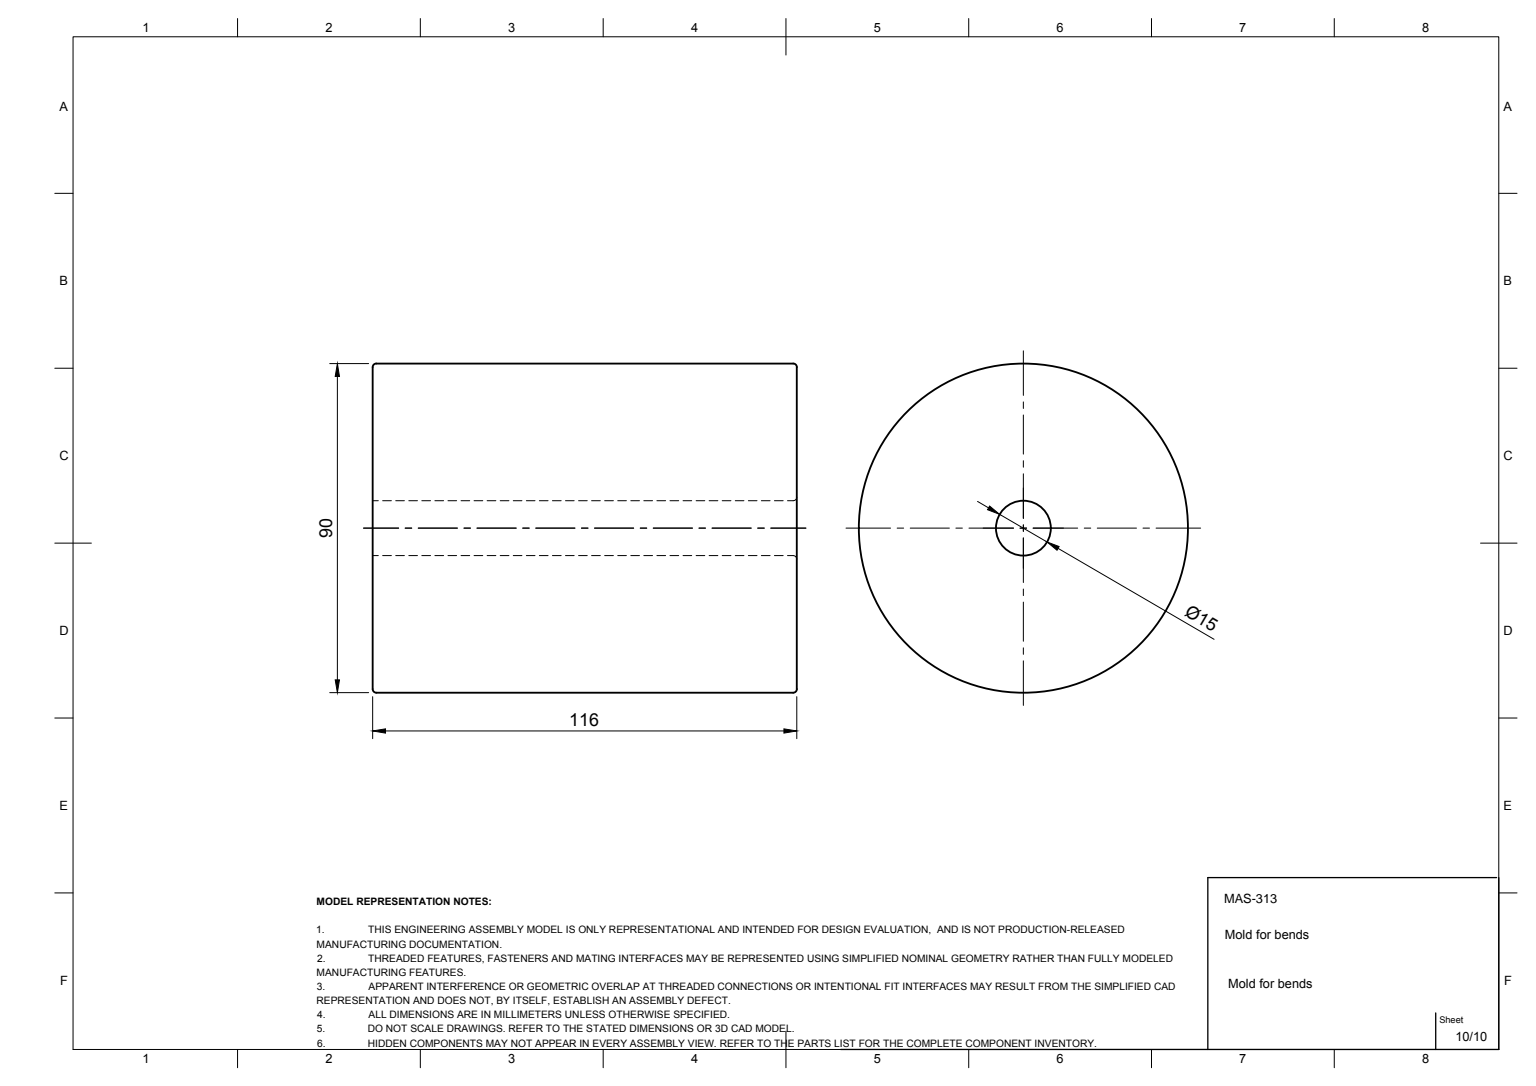
ISO-10303-21;
HEADER;
FILE_DESCRIPTION (('STEP AP214'),
    '1' );
FILE_NAME ('Mold for bends.step',
    '2026-10-06T09:36:00',
    ( '' ),
    ( '' ),
    'SwSTEP 2.0',
    'SolidWorks 2025',
    '' );
FILE_SCHEMA (( 'AUTOMOTIVE_DESIGN' ));
ENDSEC;

DATA;
#10=CIRCLE ( 'NONE', #8517, 8.500000000000007105 ) ;
#23=SHAPE_DEFINITION_REPRESENTATION ( #9502, #690 ) ;
#32=TOROIDAL_SURFACE ( 'NONE', #418, 8.500000000000007105, 1.000000000000000000 ) ;
#48=CARTESIAN_POINT ( 'NONE',  ( 7.653191805780027529E-16, 139.9999999999999716, -126.4213562373094959 ) ) ;
#147=VECTOR ( 'NONE', #6691, 1000.000000000000000 ) ;
#240=ORIENTED_EDGE ( 'NONE', *, *, #4269, .F. ) ;
#312=DIRECTION ( 'NONE',  ( -1.000000000000000000, 0.000000000000000000, 0.000000000000000000 ) ) ;
#318=DIRECTION ( 'NONE',  ( -3.061276722312011504E-17, 1.000000000000000000, 0.000000000000000000 ) ) ;
#327=ORIENTED_EDGE ( 'NONE', *, *, #355, .T. ) ;
#331=DIRECTION ( 'NONE',  ( 1.000000000000000000, 0.000000000000000000, 1.224646799147353207E-16 ) ) ;
#353=DIRECTION ( 'NONE',  ( -0.000000000000000000, -1.000000000000000000, 0.000000000000000000 ) ) ;
#355=EDGE_CURVE ( 'NONE', #1262, #3617, #2145, .T. ) ;
#418=AXIS2_PLACEMENT_3D ( 'NONE', #4659, #2540, #5635 ) ;
#434=EDGE_LOOP ( 'NONE', ( #6079, #8343 ) ) ;
#441=CARTESIAN_POINT ( 'NONE',  ( -8.500000000000003553, 24.00000000000002132, -126.4213562373094959 ) ) ;
#481=VERTEX_POINT ( 'NONE', #1901 ) ;
#500=( GEOMETRIC_REPRESENTATION_CONTEXT ( 3 ) GLOBAL_UNCERTAINTY_ASSIGNED_CONTEXT ( ( #6769 ) ) GLOBAL_UNIT_ASSIGNED_CONTEXT ( ( #4246, #9639, #11099 ) ) REPRESENTATION_CONTEXT ( 'NONE', 'WORKASPACE' ) );
#522=DIRECTION ( 'NONE',  ( 0.000000000000000000, 0.000000000000000000, 1.000000000000000000 ) ) ;
#524=TOROIDAL_SURFACE ( 'NONE', #1147, 44.00000000000000711, 1.000000000000000000 ) ;
#548=AXIS2_PLACEMENT_3D ( 'NONE', #8993, #5805, #1125 ) ;
#549=DIRECTION ( 'NONE',  ( -1.000000000000000000, -3.061276722312011504E-17, 0.000000000000000000 ) ) ;
#576=ORIENTED_EDGE ( 'NONE', *, *, #988, .T. ) ;
#635=EDGE_CURVE ( 'NONE', #11444, #3617, #5553, .T. ) ;
#690=SHAPE_REPRESENTATION ( 'Mold for bends', ( #11957 ), #500 ) ;
#704=ADVANCED_FACE ( 'NONE', ( #5459, #10101 ), #8326, .T. ) ;
#711=DIRECTION ( 'NONE',  ( 0.000000000000000000, 1.000000000000000000, -0.000000000000000000 ) ) ;
#724=EDGE_CURVE ( 'NONE', #3617, #11444, #6728, .T. ) ;
#782=EDGE_CURVE ( 'NONE', #9741, #2455, #10, .T. ) ;
#829=ORIENTED_EDGE ( 'NONE', *, *, #8003, .T. ) ;
#856=DIRECTION ( 'NONE',  ( 0.000000000000000000, 0.000000000000000000, 1.000000000000000000 ) ) ;
#867=VERTEX_POINT ( 'NONE', #1574 ) ;
#947=ORIENTED_EDGE ( 'NONE', *, *, #1332, .F. ) ;
#982=( GEOMETRIC_REPRESENTATION_CONTEXT ( 3 ) GLOBAL_UNCERTAINTY_ASSIGNED_CONTEXT ( ( #7947 ) ) GLOBAL_UNIT_ASSIGNED_CONTEXT ( ( #4651, #9582, #8536 ) ) REPRESENTATION_CONTEXT ( 'NONE', 'WORKASPACE' ) );
#988=EDGE_CURVE ( 'NONE', #6938, #1262, #2405, .T. ) ;
#1019=DIRECTION ( 'NONE',  ( -1.000000000000000000, 0.000000000000000000, 0.000000000000000000 ) ) ;
#1030=ADVANCED_FACE ( 'NONE', ( #11648 ), #2322, .T. ) ;
#1045=ORIENTED_EDGE ( 'NONE', *, *, #1101, .F. ) ;
#1101=EDGE_CURVE ( 'NONE', #3987, #7340, #5116, .T. ) ;
#1113=FACE_OUTER_BOUND ( 'NONE', #10754, .T. ) ;
#1125=DIRECTION ( 'NONE',  ( -1.000000000000000000, 0.000000000000000000, 0.000000000000000000 ) ) ;
#1147=AXIS2_PLACEMENT_3D ( 'NONE', #9115, #6335, #522 ) ;
#1178=AXIS2_PLACEMENT_3D ( 'NONE', #5862, #5742, #8485 ) ;
#1228=DIRECTION ( 'NONE',  ( 1.000000000000000000, 0.000000000000000000, 0.000000000000000000 ) ) ;
#1262=VERTEX_POINT ( 'NONE', #6358 ) ;
#1307=LINE ( 'NONE', #6922, #12091 ) ;
#1332=EDGE_CURVE ( 'NONE', #4924, #2829, #4976, .T. ) ;
#1369=CARTESIAN_POINT ( 'NONE',  ( 4.285787411236815022E-15, 24.00000000000001776, -126.4213562373094959 ) ) ;
#1390=EDGE_CURVE ( 'NONE', #7340, #3987, #8949, .T. ) ;
#1438=ORIENTED_EDGE ( 'NONE', *, *, #5723, .F. ) ;
#1533=CARTESIAN_POINT ( 'NONE',  ( 4.255174644013695128E-15, 25.00000000000002132, -126.4213562373094959 ) ) ;
#1540=ORIENTED_EDGE ( 'NONE', *, *, #9548, .T. ) ;
#1574=CARTESIAN_POINT ( 'NONE',  ( -7.500000000000007105, 139.9999999999999716, -126.4213562373094959 ) ) ;
#1577=CARTESIAN_POINT ( 'NONE',  ( 4.285787411236815022E-15, 24.00000000000001776, -126.4213562373094959 ) ) ;
#1580=DIRECTION ( 'NONE',  ( -1.000000000000000000, 0.000000000000000000, 0.000000000000000000 ) ) ;
#1589=VERTEX_POINT ( 'NONE', #7656 ) ;
#1600=CARTESIAN_POINT ( 'NONE',  ( 8.500000000000010658, 25.00000000000002132, -126.4213562373094959 ) ) ;
#1811=AXIS2_PLACEMENT_3D ( 'NONE', #11030, #711, #11893 ) ;
#1829=DIRECTION ( 'NONE',  ( -3.061276722312011504E-17, 1.000000000000000000, 0.000000000000000000 ) ) ;
#1874=AXIS2_PLACEMENT_3D ( 'NONE', #1577, #6860, #4490 ) ;
#1901=CARTESIAN_POINT ( 'NONE',  ( -7.500000000000004441, 25.00000000000002132, -126.4213562373094959 ) ) ;
#1945=DIRECTION ( 'NONE',  ( -1.000000000000000000, -3.061276722312011504E-17, 0.000000000000000000 ) ) ;
#1952=CIRCLE ( 'NONE', #11230, 7.500000000000007994 ) ;
#1973=CLOSED_SHELL ( 'NONE', ( #1030, #2315, #10373, #8644, #12238, #11825, #10263, #3894, #704, #12063, #5255, #9325 ) ) ;
#1981=DIRECTION ( 'NONE',  ( 0.000000000000000000, 1.000000000000000000, -0.000000000000000000 ) ) ;
#1987=DIRECTION ( 'NONE',  ( 3.061276722312011504E-17, -1.000000000000000000, -0.000000000000000000 ) ) ;
#2023=CARTESIAN_POINT ( 'NONE',  ( 45.00000000000000711, 138.9999999999999716, -126.4213562373094959 ) ) ;
#2039=FILL_AREA_STYLE_COLOUR ( '', #5518 ) ;
#2071=DIRECTION ( 'NONE',  ( 0.000000000000000000, 0.000000000000000000, 1.000000000000000000 ) ) ;
#2089=AXIS2_PLACEMENT_3D ( 'NONE', #10446, #1987, #6861 ) ;
#2145=LINE ( 'NONE', #2894, #10261 ) ;
#2315=ADVANCED_FACE ( 'NONE', ( #11225 ), #10336, .T. ) ;
#2322=TOROIDAL_SURFACE ( 'NONE', #10803, 44.00000000000000711, 1.000000000000000000 ) ;
#2331=CARTESIAN_POINT ( 'NONE',  ( 4.255174644013695128E-15, 25.00000000000002132, -126.4213562373094959 ) ) ;
#2343=APPLICATION_CONTEXT ( 'automotive_design' ) ;
#2405=CIRCLE ( 'NONE', #7742, 45.00000000000001421 ) ;
#2455=VERTEX_POINT ( 'NONE', #7714 ) ;
#2495=DIRECTION ( 'NONE',  ( -1.000000000000000000, 0.000000000000000000, 0.000000000000000000 ) ) ;
#2501=EDGE_LOOP ( 'NONE', ( #947, #7426, #10048, #10580, #9332 ) ) ;
#2540=DIRECTION ( 'NONE',  ( -3.061276722312011504E-17, 1.000000000000000000, 0.000000000000000000 ) ) ;
#2560=ORIENTED_EDGE ( 'NONE', *, *, #6918, .F. ) ;
#2614=DIRECTION ( 'NONE',  ( -3.061276722312011504E-17, 1.000000000000000000, 0.000000000000000000 ) ) ;
#2677=AXIS2_PLACEMENT_3D ( 'NONE', #2690, #5717, #12164 ) ;
#2690=CARTESIAN_POINT ( 'NONE',  ( 7.653191805780027529E-16, 138.9999999999999716, -126.4213562373094959 ) ) ;
#2761=CARTESIAN_POINT ( 'NONE',  ( -7.500000000000011546, 267.2792206135785591, -126.4213562373094959 ) ) ;
#2825=PRODUCT_DEFINITION_CONTEXT ( 'detailed design', #2343, 'design' ) ;
#2829=VERTEX_POINT ( 'NONE', #2023 ) ;
#2894=CARTESIAN_POINT ( 'NONE',  ( -45.00000000000000711, 267.2792206135785591, -126.4213562373094959 ) ) ;
#2895=ORIENTED_EDGE ( 'NONE', *, *, #5993, .T. ) ;
#2931=CARTESIAN_POINT ( 'NONE',  ( 45.00000000000000711, 267.2792206135785591, -126.4213562373094959 ) ) ;
#3020=AXIS2_PLACEMENT_3D ( 'NONE', #4543, #11151, #3464 ) ;
#3023=CARTESIAN_POINT ( 'NONE',  ( 7.653191805780027529E-16, 139.9999999999999716, -126.4213562373094959 ) ) ;
#3031=ORIENTED_EDGE ( 'NONE', *, *, #8003, .F. ) ;
#3059=PRODUCT_CONTEXT ( 'NONE', #4004, 'mechanical' ) ;
#3073=ORIENTED_EDGE ( 'NONE', *, *, #10401, .T. ) ;
#3078=EDGE_CURVE ( 'NONE', #7692, #2455, #9370, .T. ) ;
#3092=CARTESIAN_POINT ( 'NONE',  ( 7.653191805780027529E-16, 139.9999999999999716, -82.42135623730948168 ) ) ;
#3120=CARTESIAN_POINT ( 'NONE',  ( 6.153765096826357259E-15, 138.9999999999999716, -170.4213562373095101 ) ) ;
#3140=DIRECTION ( 'NONE',  ( 0.000000000000000000, 0.000000000000000000, 1.000000000000000000 ) ) ;
#3146=ORIENTED_EDGE ( 'NONE', *, *, #7457, .T. ) ;
#3237=DIRECTION ( 'NONE',  ( -1.000000000000000000, 0.000000000000000000, 0.000000000000000000 ) ) ;
#3310=CIRCLE ( 'NONE', #548, 7.500000000000007994 ) ;
#3323=ORIENTED_EDGE ( 'NONE', *, *, #9548, .F. ) ;
#3423=DIRECTION ( 'NONE',  ( -3.061276722312011504E-17, 1.000000000000000000, 0.000000000000000000 ) ) ;
#3464=DIRECTION ( 'NONE',  ( 0.000000000000000000, 0.000000000000000000, 1.000000000000000000 ) ) ;
#3471=FACE_OUTER_BOUND ( 'NONE', #5847, .T. ) ;
#3482=ORIENTED_EDGE ( 'NONE', *, *, #12070, .F. ) ;
#3535=CARTESIAN_POINT ( 'NONE',  ( 4.255174644013695128E-15, 25.00000000000002132, -126.4213562373094959 ) ) ;
#3617=VERTEX_POINT ( 'NONE', #8789 ) ;
#3620=AXIS2_PLACEMENT_3D ( 'NONE', #3023, #1981, #3140 ) ;
#3888=AXIS2_PLACEMENT_3D ( 'NONE', #9058, #3423, #8139 ) ;
#3894=ADVANCED_FACE ( 'NONE', ( #6554 ), #10320, .F. ) ;
#3906=ORIENTED_EDGE ( 'NONE', *, *, #9393, .T. ) ;
#3942=MANIFOLD_SOLID_BREP ( 'Fillet8', #1973 ) ;
#3987=VERTEX_POINT ( 'NONE', #4993 ) ;
#4001=ORIENTED_EDGE ( 'NONE', *, *, #10401, .F. ) ;
#4004=APPLICATION_CONTEXT ( 'automotive_design' ) ;
#4014=DIRECTION ( 'NONE',  ( 0.000000000000000000, 0.000000000000000000, 1.000000000000000000 ) ) ;
#4041=CARTESIAN_POINT ( 'NONE',  ( 45.00000000000001421, 25.00000000000002132, -126.4213562373094959 ) ) ;
#4062=TOROIDAL_SURFACE ( 'NONE', #2677, 44.00000000000000711, 1.000000000000000000 ) ;
#4196=EDGE_LOOP ( 'NONE', ( #5886, #2895, #6082, #829, #8818 ) ) ;
#4246=( LENGTH_UNIT ( ) NAMED_UNIT ( * ) SI_UNIT ( .MILLI., .METRE. ) );
#4260=EDGE_CURVE ( 'NONE', #7692, #481, #1952, .T. ) ;
#4269=EDGE_CURVE ( 'NONE', #481, #7692, #3310, .T. ) ;
#4384=ORIENTED_EDGE ( 'NONE', *, *, #6373, .F. ) ;
#4425=CIRCLE ( 'NONE', #10540, 44.00000000000000711 ) ;
#4490=DIRECTION ( 'NONE',  ( -1.000000000000000000, 0.000000000000000000, 0.000000000000000000 ) ) ;
#4543=CARTESIAN_POINT ( 'NONE',  ( 7.653191805780027529E-16, 138.9999999999999716, -126.4213562373094959 ) ) ;
#4584=DIRECTION ( 'NONE',  ( -1.224646799147353207E-16, -3.748982739283705415E-33, 1.000000000000000000 ) ) ;
#4646=ORIENTED_EDGE ( 'NONE', *, *, #724, .T. ) ;
#4651=( LENGTH_UNIT ( ) NAMED_UNIT ( * ) SI_UNIT ( .MILLI., .METRE. ) );
#4659=CARTESIAN_POINT ( 'NONE',  ( 4.255174644013695128E-15, 25.00000000000002132, -126.4213562373094959 ) ) ;
#4691=DIRECTION ( 'NONE',  ( 0.000000000000000000, 1.000000000000000000, -0.000000000000000000 ) ) ;
#4843=CARTESIAN_POINT ( 'NONE',  ( 7.653191805780027529E-16, 138.9999999999999716, -126.4213562373094959 ) ) ;
#4877=DIRECTION ( 'NONE',  ( 3.061276722312011504E-17, -1.000000000000000000, -0.000000000000000000 ) ) ;
#4924=VERTEX_POINT ( 'NONE', #11567 ) ;
#4976=CIRCLE ( 'NONE', #5507, 45.00000000000001421 ) ;
#4993=CARTESIAN_POINT ( 'NONE',  ( 6.214997436783724833E-15, 139.9999999999999716, -170.4213562373095101 ) ) ;
#5116=CIRCLE ( 'NONE', #5515, 44.00000000000001421 ) ;
#5124=DIRECTION ( 'NONE',  ( -0.000000000000000000, -1.000000000000000000, 0.000000000000000000 ) ) ;
#5159=DIRECTION ( 'NONE',  ( 3.061276722312011504E-17, -1.000000000000000000, -0.000000000000000000 ) ) ;
#5165=DIRECTION ( 'NONE',  ( -1.000000000000000000, 0.000000000000000000, 0.000000000000000000 ) ) ;
#5212=CYLINDRICAL_SURFACE ( 'NONE', #10574, 45.00000000000000711 ) ;
#5217=EDGE_LOOP ( 'NONE', ( #5959, #5712 ) ) ;
#5218=FACE_OUTER_BOUND ( 'NONE', #2501, .T. ) ;
#5241=AXIS2_PLACEMENT_3D ( 'NONE', #8286, #5352, #8219 ) ;
#5255=ADVANCED_FACE ( 'NONE', ( #3471 ), #32, .T. ) ;
#5300=STYLED_ITEM ( 'NONE', ( #8594 ), #3942 ) ;
#5352=DIRECTION ( 'NONE',  ( -1.224646799147353207E-16, -3.748982739283705415E-33, 1.000000000000000000 ) ) ;
#5372=ORIENTED_EDGE ( 'NONE', *, *, #4260, .F. ) ;
#5394=CARTESIAN_POINT ( 'NONE',  ( 4.285787411236815022E-15, 24.00000000000001776, -126.4213562373094959 ) ) ;
#5405=EDGE_CURVE ( 'NONE', #1589, #7692, #1307, .T. ) ;
#5423=ORIENTED_EDGE ( 'NONE', *, *, #3078, .F. ) ;
#5459=FACE_OUTER_BOUND ( 'NONE', #434, .T. ) ;
#5507=AXIS2_PLACEMENT_3D ( 'NONE', #11623, #353, #4014 ) ;
#5515=AXIS2_PLACEMENT_3D ( 'NONE', #48, #5678, #7600 ) ;
#5518=COLOUR_RGB ( '', 0.40784314, 0.44705882, 0.49803922) ;
#5553=CIRCLE ( 'NONE', #7127, 45.00000000000000711 ) ;
#5603=EDGE_CURVE ( 'NONE', #867, #1589, #11696, .T. ) ;
#5623=CIRCLE ( 'NONE', #9175, 8.500000000000007105 ) ;
#5635=DIRECTION ( 'NONE',  ( -1.000000000000000000, -3.061276722312011504E-17, 0.000000000000000000 ) ) ;
#5637=VECTOR ( 'NONE', #8513, 1000.000000000000000 ) ;
#5678=DIRECTION ( 'NONE',  ( 0.000000000000000000, 1.000000000000000000, -0.000000000000000000 ) ) ;
#5712=ORIENTED_EDGE ( 'NONE', *, *, #5603, .F. ) ;
#5717=DIRECTION ( 'NONE',  ( 0.000000000000000000, 1.000000000000000000, -0.000000000000000000 ) ) ;
#5723=EDGE_CURVE ( 'NONE', #4924, #3987, #9917, .T. ) ;
#5742=DIRECTION ( 'NONE',  ( 3.061276722312011504E-17, -1.000000000000000000, -0.000000000000000000 ) ) ;
#5805=DIRECTION ( 'NONE',  ( 3.061276722312011504E-17, -1.000000000000000000, -0.000000000000000000 ) ) ;
#5826=CARTESIAN_POINT ( 'NONE',  ( -8.500000000000003553, 25.00000000000002132, -126.4213562373094959 ) ) ;
#5847=EDGE_LOOP ( 'NONE', ( #5423, #240, #1540, #10764 ) ) ;
#5862=CARTESIAN_POINT ( 'NONE',  ( -3.161662739628749519E-15, 267.2792206135785591, -126.4213562373094959 ) ) ;
#5886=ORIENTED_EDGE ( 'NONE', *, *, #355, .F. ) ;
#5959=ORIENTED_EDGE ( 'NONE', *, *, #7571, .F. ) ;
#5993=EDGE_CURVE ( 'NONE', #1262, #4924, #8917, .T. ) ;
#6079=ORIENTED_EDGE ( 'NONE', *, *, #1390, .T. ) ;
#6082=ORIENTED_EDGE ( 'NONE', *, *, #1332, .T. ) ;
#6106=CARTESIAN_POINT ( 'NONE',  ( 7.347064133548826625E-16, 139.9999999999999716, -126.4213562373094959 ) ) ;
#6116=CARTESIAN_POINT ( 'NONE',  ( 7.653191805780027529E-16, 138.9999999999999716, -126.4213562373094959 ) ) ;
#6127=DIRECTION ( 'NONE',  ( 3.061276722312011504E-17, -1.000000000000000000, -0.000000000000000000 ) ) ;
#6202=ORIENTED_EDGE ( 'NONE', *, *, #6918, .T. ) ;
#6214=CIRCLE ( 'NONE', #7411, 7.500000000000007105 ) ;
#6254=ORIENTED_EDGE ( 'NONE', *, *, #4260, .T. ) ;
#6261=CIRCLE ( 'NONE', #9010, 1.000000000000000888 ) ;
#6319=EDGE_CURVE ( 'NONE', #6938, #7340, #8578, .T. ) ;
#6335=DIRECTION ( 'NONE',  ( 0.000000000000000000, 1.000000000000000000, -0.000000000000000000 ) ) ;
#6358=CARTESIAN_POINT ( 'NONE',  ( -45.00000000000000711, 138.9999999999999716, -126.4213562373094959 ) ) ;
#6373=EDGE_CURVE ( 'NONE', #8852, #6960, #4425, .T. ) ;
#6386=CARTESIAN_POINT ( 'NONE',  ( 7.500000000000012434, 25.00000000000002132, -126.4213562373094959 ) ) ;
#6503=ORIENTED_EDGE ( 'NONE', *, *, #988, .F. ) ;
#6554=FACE_OUTER_BOUND ( 'NONE', #8057, .T. ) ;
#6691=DIRECTION ( 'NONE',  ( 3.061276722312011504E-17, -1.000000000000000000, -0.000000000000000000 ) ) ;
#6702=ORIENTED_EDGE ( 'NONE', *, *, #5405, .T. ) ;
#6728=CIRCLE ( 'NONE', #9696, 45.00000000000000711 ) ;
#6769=UNCERTAINTY_MEASURE_WITH_UNIT (LENGTH_MEASURE( 1.000000000000000082E-05 ), #4246, 'distance_accuracy_value', 'NONE');
#6783=AXIS2_PLACEMENT_3D ( 'NONE', #8106, #8895, #6990 ) ;
#6860=DIRECTION ( 'NONE',  ( 3.061276722312011504E-17, -1.000000000000000000, -0.000000000000000000 ) ) ;
#6861=DIRECTION ( 'NONE',  ( 1.000000000000000000, 0.000000000000000000, 0.000000000000000000 ) ) ;
#6898=EDGE_LOOP ( 'NONE', ( #4384, #3906, #7268, #4001 ) ) ;
#6907=CYLINDRICAL_SURFACE ( 'NONE', #8671, 7.500000000000007994 ) ;
#6918=EDGE_CURVE ( 'NONE', #6960, #8852, #8957, .T. ) ;
#6922=CARTESIAN_POINT ( 'NONE',  ( 7.500000000000005329, 267.2792206135785591, -126.4213562373094959 ) ) ;
#6938=VERTEX_POINT ( 'NONE', #7142 ) ;
#6960=VERTEX_POINT ( 'NONE', #10906 ) ;
#6990=DIRECTION ( 'NONE',  ( 0.000000000000000000, 0.000000000000000000, 1.000000000000000000 ) ) ;
#7006=EDGE_LOOP ( 'NONE', ( #7931, #3146 ) ) ;
#7062=ORIENTED_EDGE ( 'NONE', *, *, #635, .F. ) ;
#7127=AXIS2_PLACEMENT_3D ( 'NONE', #7950, #11722, #3237 ) ;
#7142=CARTESIAN_POINT ( 'NONE',  ( 7.653191805780027529E-16, 138.9999999999999716, -81.42135623730948168 ) ) ;
#7199=DIRECTION ( 'NONE',  ( -3.061276722312011504E-17, 1.000000000000000000, 0.000000000000000000 ) ) ;
#7233=CARTESIAN_POINT ( 'NONE',  ( 4.255174644013695128E-15, 25.00000000000002132, -126.4213562373094959 ) ) ;
#7266=SHAPE_REPRESENTATION_RELATIONSHIP ( 'NONE' , 'NONE' ,  #690, #8261 ) ;
#7268=ORIENTED_EDGE ( 'NONE', *, *, #724, .F. ) ;
#7321=ORIENTED_EDGE ( 'NONE', *, *, #9393, .F. ) ;
#7340=VERTEX_POINT ( 'NONE', #3092 ) ;
#7411=AXIS2_PLACEMENT_3D ( 'NONE', #6106, #11222, #10095 ) ;
#7417=EDGE_LOOP ( 'NONE', ( #6202, #11645 ) ) ;
#7426=ORIENTED_EDGE ( 'NONE', *, *, #5723, .T. ) ;
#7430=CIRCLE ( 'NONE', #8439, 1.000000000000000888 ) ;
#7453=TOROIDAL_SURFACE ( 'NONE', #8228, 44.00000000000000711, 1.000000000000000000 ) ;
#7457=EDGE_CURVE ( 'NONE', #2455, #9741, #5623, .T. ) ;
#7481=DIRECTION ( 'NONE',  ( 1.000000000000000000, 0.000000000000000000, 0.000000000000000000 ) ) ;
#7542=SURFACE_STYLE_FILL_AREA ( #10379 ) ;
#7571=EDGE_CURVE ( 'NONE', #1589, #867, #6214, .T. ) ;
#7600=DIRECTION ( 'NONE',  ( 0.000000000000000000, 0.000000000000000000, 1.000000000000000000 ) ) ;
#7605=SURFACE_STYLE_USAGE ( .BOTH. , #10506 ) ;
#7608=FACE_OUTER_BOUND ( 'NONE', #4196, .T. ) ;
#7616=AXIS2_PLACEMENT_3D ( 'NONE', #6116, #5124, #7852 ) ;
#7638=LINE ( 'NONE', #2761, #5637 ) ;
#7656=CARTESIAN_POINT ( 'NONE',  ( 7.500000000000008882, 139.9999999999999716, -126.4213562373094959 ) ) ;
#7692=VERTEX_POINT ( 'NONE', #6386 ) ;
#7714=CARTESIAN_POINT ( 'NONE',  ( 8.500000000000010658, 24.00000000000002132, -126.4213562373094959 ) ) ;
#7731=DIRECTION ( 'NONE',  ( -1.000000000000000000, 0.000000000000000000, 0.000000000000000000 ) ) ;
#7742=AXIS2_PLACEMENT_3D ( 'NONE', #4843, #8621, #2071 ) ;
#7827=CIRCLE ( 'NONE', #5241, 1.000000000000000888 ) ;
#7852=DIRECTION ( 'NONE',  ( 0.000000000000000000, 0.000000000000000000, 1.000000000000000000 ) ) ;
#7859=DIRECTION ( 'NONE',  ( 3.061276722312011504E-17, -1.000000000000000000, -0.000000000000000000 ) ) ;
#7931=ORIENTED_EDGE ( 'NONE', *, *, #782, .T. ) ;
#7947=UNCERTAINTY_MEASURE_WITH_UNIT (LENGTH_MEASURE( 1.000000000000000082E-05 ), #4651, 'distance_accuracy_value', 'NONE');
#7950=CARTESIAN_POINT ( 'NONE',  ( 4.255174644013695128E-15, 25.00000000000002132, -126.4213562373094959 ) ) ;
#7955=DIRECTION ( 'NONE',  ( 1.000000000000000000, 0.000000000000000000, 0.000000000000000000 ) ) ;
#8003=EDGE_CURVE ( 'NONE', #2829, #11444, #11393, .T. ) ;
#8057=EDGE_LOOP ( 'NONE', ( #3482, #10997, #6702, #6254 ) ) ;
#8073=DIRECTION ( 'NONE',  ( 1.000000000000000000, 0.000000000000000000, 0.000000000000000000 ) ) ;
#8106=CARTESIAN_POINT ( 'NONE',  ( 7.653191805780027529E-16, 138.9999999999999716, -82.42135623730948168 ) ) ;
#8107=CARTESIAN_POINT ( 'NONE',  ( 44.00000000000001421, 24.00000000000001776, -126.4213562373094959 ) ) ;
#8139=DIRECTION ( 'NONE',  ( -1.000000000000000000, -3.061276722312011504E-17, 0.000000000000000000 ) ) ;
#8197=DIRECTION ( 'NONE',  ( -1.000000000000000000, 0.000000000000000000, 0.000000000000000000 ) ) ;
#8219=DIRECTION ( 'NONE',  ( 1.000000000000000000, 0.000000000000000000, 0.000000000000000000 ) ) ;
#8228=AXIS2_PLACEMENT_3D ( 'NONE', #1533, #10188, #10121 ) ;
#8261=ADVANCED_BREP_SHAPE_REPRESENTATION ( '', ( #3942, #11957 ), #500 ) ;
#8286=CARTESIAN_POINT ( 'NONE',  ( 44.00000000000001421, 25.00000000000002132, -126.4213562373094959 ) ) ;
#8326=PLANE ( 'NONE',  #1811 ) ;
#8343=ORIENTED_EDGE ( 'NONE', *, *, #1101, .T. ) ;
#8439=AXIS2_PLACEMENT_3D ( 'NONE', #5826, #9603, #1019 ) ;
#8485=DIRECTION ( 'NONE',  ( 1.000000000000000000, 0.000000000000000000, 0.000000000000000000 ) ) ;
#8513=DIRECTION ( 'NONE',  ( 3.061276722312011504E-17, -1.000000000000000000, -0.000000000000000000 ) ) ;
#8517=AXIS2_PLACEMENT_3D ( 'NONE', #5394, #1829, #8197 ) ;
#8536=( NAMED_UNIT ( * ) SI_UNIT ( $, .STERADIAN. ) SOLID_ANGLE_UNIT ( ) );
#8545=AXIS2_PLACEMENT_3D ( 'NONE', #3120, #331, #10722 ) ;
#8578=CIRCLE ( 'NONE', #6783, 1.000000000000000888 ) ;
#8594=PRESENTATION_STYLE_ASSIGNMENT (( #7605 ) ) ;
#8602=ORIENTED_EDGE ( 'NONE', *, *, #3078, .T. ) ;
#8621=DIRECTION ( 'NONE',  ( -0.000000000000000000, -1.000000000000000000, 0.000000000000000000 ) ) ;
#8644=ADVANCED_FACE ( 'NONE', ( #1113 ), #6907, .F. ) ;
#8671=AXIS2_PLACEMENT_3D ( 'NONE', #10555, #9808, #1228 ) ;
#8757=DIRECTION ( 'NONE',  ( 3.061276722312011504E-17, -1.000000000000000000, -0.000000000000000000 ) ) ;
#8776=AXIS2_PLACEMENT_3D ( 'NONE', #1600, #4584, #7481 ) ;
#8789=CARTESIAN_POINT ( 'NONE',  ( -45.00000000000000000, 25.00000000000002132, -126.4213562373094959 ) ) ;
#8817=FACE_OUTER_BOUND ( 'NONE', #10835, .T. ) ;
#8818=ORIENTED_EDGE ( 'NONE', *, *, #635, .T. ) ;
#8852=VERTEX_POINT ( 'NONE', #8107 ) ;
#8895=DIRECTION ( 'NONE',  ( -1.000000000000000000, 0.000000000000000000, 0.000000000000000000 ) ) ;
#8917=CIRCLE ( 'NONE', #3020, 45.00000000000001421 ) ;
#8949=CIRCLE ( 'NONE', #3620, 44.00000000000001421 ) ;
#8957=CIRCLE ( 'NONE', #1874, 44.00000000000000711 ) ;
#8991=DIRECTION ( 'NONE',  ( -0.000000000000000000, 0.000000000000000000, -1.000000000000000000 ) ) ;
#8993=CARTESIAN_POINT ( 'NONE',  ( 4.255174644013695128E-15, 25.00000000000002132, -126.4213562373094959 ) ) ;
#9010=AXIS2_PLACEMENT_3D ( 'NONE', #9870, #8991, #1580 ) ;
#9048=CARTESIAN_POINT ( 'NONE',  ( 0.000000000000000000, 0.000000000000000000, 0.000000000000000000 ) ) ;
#9058=CARTESIAN_POINT ( 'NONE',  ( 4.285787411236815022E-15, 24.00000000000001776, -126.4213562373094959 ) ) ;
#9095=ORIENTED_EDGE ( 'NONE', *, *, #7571, .T. ) ;
#9115=CARTESIAN_POINT ( 'NONE',  ( 7.653191805780027529E-16, 138.9999999999999716, -126.4213562373094959 ) ) ;
#9175=AXIS2_PLACEMENT_3D ( 'NONE', #11270, #11506, #7731 ) ;
#9325=ADVANCED_FACE ( 'NONE', ( #10416 ), #7453, .T. ) ;
#9332=ORIENTED_EDGE ( 'NONE', *, *, #11879, .F. ) ;
#9370=CIRCLE ( 'NONE', #8776, 1.000000000000000888 ) ;
#9393=EDGE_CURVE ( 'NONE', #8852, #11444, #7827, .T. ) ;
#9502=PRODUCT_DEFINITION_SHAPE ( 'NONE', 'NONE',  #10256 ) ;
#9548=EDGE_CURVE ( 'NONE', #481, #9741, #7430, .T. ) ;
#9582=( NAMED_UNIT ( * ) PLANE_ANGLE_UNIT ( ) SI_UNIT ( $, .RADIAN. ) );
#9603=DIRECTION ( 'NONE',  ( -0.000000000000000000, 0.000000000000000000, -1.000000000000000000 ) ) ;
#9639=( NAMED_UNIT ( * ) PLANE_ANGLE_UNIT ( ) SI_UNIT ( $, .RADIAN. ) );
#9696=AXIS2_PLACEMENT_3D ( 'NONE', #3535, #7199, #2495 ) ;
#9741=VERTEX_POINT ( 'NONE', #441 ) ;
#9808=DIRECTION ( 'NONE',  ( 3.061276722312011504E-17, -1.000000000000000000, -0.000000000000000000 ) ) ;
#9818=EDGE_LOOP ( 'NONE', ( #5372, #8602, #11597, #3323 ) ) ;
#9865=CARTESIAN_POINT ( 'NONE',  ( -3.161662739628749519E-15, 267.2792206135785591, -126.4213562373094959 ) ) ;
#9870=CARTESIAN_POINT ( 'NONE',  ( -44.00000000000000000, 25.00000000000002132, -126.4213562373094959 ) ) ;
#9917=CIRCLE ( 'NONE', #8545, 1.000000000000000888 ) ;
#9991=PRODUCT_DEFINITION_FORMATION_WITH_SPECIFIED_SOURCE ( 'ANY', '', #10588, .NOT_KNOWN. ) ;
#10048=ORIENTED_EDGE ( 'NONE', *, *, #1390, .F. ) ;
#10095=DIRECTION ( 'NONE',  ( 0.000000000000000000, 0.000000000000000000, 1.000000000000000000 ) ) ;
#10101=FACE_BOUND ( 'NONE', #5217, .T. ) ;
#10111=PLANE ( 'NONE',  #3888 ) ;
#10121=DIRECTION ( 'NONE',  ( -1.000000000000000000, -3.061276722312011504E-17, 0.000000000000000000 ) ) ;
#10139=AXIS2_PLACEMENT_3D ( 'NONE', #12086, #2614, #1945 ) ;
#10171=FACE_OUTER_BOUND ( 'NONE', #12011, .T. ) ;
#10188=DIRECTION ( 'NONE',  ( -3.061276722312011504E-17, 1.000000000000000000, 0.000000000000000000 ) ) ;
#10256=PRODUCT_DEFINITION ( 'UNKNOWN', '', #9991, #2825 ) ;
#10261=VECTOR ( 'NONE', #8757, 1000.000000000000000 ) ;
#10263=ADVANCED_FACE ( 'NONE', ( #11966, #11486 ), #10111, .F. ) ;
#10276=ORIENTED_EDGE ( 'NONE', *, *, #11879, .T. ) ;
#10304=AXIS2_PLACEMENT_3D ( 'NONE', #10424, #4691, #856 ) ;
#10320=CYLINDRICAL_SURFACE ( 'NONE', #1178, 7.500000000000007994 ) ;
#10336=TOROIDAL_SURFACE ( 'NONE', #10139, 8.500000000000007105, 1.000000000000000000 ) ;
#10373=ADVANCED_FACE ( 'NONE', ( #5218 ), #524, .T. ) ;
#10379=FILL_AREA_STYLE ('',( #2039 ) ) ;
#10401=EDGE_CURVE ( 'NONE', #6960, #3617, #6261, .T. ) ;
#10416=FACE_OUTER_BOUND ( 'NONE', #11322, .T. ) ;
#10424=CARTESIAN_POINT ( 'NONE',  ( 7.347064133548826625E-16, 139.9999999999999716, -126.4213562373094959 ) ) ;
#10446=CARTESIAN_POINT ( 'NONE',  ( -3.161662739628749519E-15, 267.2792206135785591, -126.4213562373094959 ) ) ;
#10506=SURFACE_SIDE_STYLE ('',( #7542 ) ) ;
#10540=AXIS2_PLACEMENT_3D ( 'NONE', #1369, #6127, #312 ) ;
#10555=CARTESIAN_POINT ( 'NONE',  ( -3.161662739628749519E-15, 267.2792206135785591, -126.4213562373094959 ) ) ;
#10574=AXIS2_PLACEMENT_3D ( 'NONE', #9865, #5159, #8073 ) ;
#10580=ORIENTED_EDGE ( 'NONE', *, *, #6319, .F. ) ;
#10588=PRODUCT ( 'Mold for bends', 'Mold for bends', '', ( #3059 ) ) ;
#10658=ORIENTED_EDGE ( 'NONE', *, *, #12070, .T. ) ;
#10722=DIRECTION ( 'NONE',  ( 1.224646799147349509E-16, 0.000000000000000000, -1.000000000000000000 ) ) ;
#10754=EDGE_LOOP ( 'NONE', ( #9095, #10658, #11628, #11743 ) ) ;
#10764=ORIENTED_EDGE ( 'NONE', *, *, #7457, .F. ) ;
#10803=AXIS2_PLACEMENT_3D ( 'NONE', #7233, #318, #549 ) ;
#10835=EDGE_LOOP ( 'NONE', ( #10276, #576, #327, #4646, #3031 ) ) ;
#10904=DIRECTION ( 'NONE',  ( 0.000000000000000000, 0.000000000000000000, 1.000000000000000000 ) ) ;
#10906=CARTESIAN_POINT ( 'NONE',  ( -44.00000000000000000, 24.00000000000001776, -126.4213562373094959 ) ) ;
#10997=ORIENTED_EDGE ( 'NONE', *, *, #5603, .T. ) ;
#11030=CARTESIAN_POINT ( 'NONE',  ( 35.00000000000000000, 139.9999999999999716, -89.68077099980384048 ) ) ;
#11097=ORIENTED_EDGE ( 'NONE', *, *, #6319, .T. ) ;
#11099=( NAMED_UNIT ( * ) SI_UNIT ( $, .STERADIAN. ) SOLID_ANGLE_UNIT ( ) );
#11151=DIRECTION ( 'NONE',  ( -0.000000000000000000, -1.000000000000000000, 0.000000000000000000 ) ) ;
#11222=DIRECTION ( 'NONE',  ( 0.000000000000000000, 1.000000000000000000, -0.000000000000000000 ) ) ;
#11225=FACE_OUTER_BOUND ( 'NONE', #9818, .T. ) ;
#11230=AXIS2_PLACEMENT_3D ( 'NONE', #2331, #4877, #5165 ) ;
#11250=MECHANICAL_DESIGN_GEOMETRIC_PRESENTATION_REPRESENTATION('',(#5300),#982);
#11270=CARTESIAN_POINT ( 'NONE',  ( 4.285787411236815022E-15, 24.00000000000001776, -126.4213562373094959 ) ) ;
#11322=EDGE_LOOP ( 'NONE', ( #7321, #2560, #3073, #7062 ) ) ;
#11373=CYLINDRICAL_SURFACE ( 'NONE', #2089, 45.00000000000000711 ) ;
#11393=LINE ( 'NONE', #2931, #147 ) ;
#11444=VERTEX_POINT ( 'NONE', #4041 ) ;
#11486=FACE_OUTER_BOUND ( 'NONE', #7417, .T. ) ;
#11506=DIRECTION ( 'NONE',  ( -3.061276722312011504E-17, 1.000000000000000000, 0.000000000000000000 ) ) ;
#11562=CIRCLE ( 'NONE', #7616, 45.00000000000001421 ) ;
#11567=CARTESIAN_POINT ( 'NONE',  ( 6.276229776741093196E-15, 138.9999999999999716, -171.4213562373095101 ) ) ;
#11597=ORIENTED_EDGE ( 'NONE', *, *, #782, .F. ) ;
#11623=CARTESIAN_POINT ( 'NONE',  ( 7.653191805780027529E-16, 138.9999999999999716, -126.4213562373094959 ) ) ;
#11628=ORIENTED_EDGE ( 'NONE', *, *, #4269, .T. ) ;
#11645=ORIENTED_EDGE ( 'NONE', *, *, #6373, .T. ) ;
#11648=FACE_OUTER_BOUND ( 'NONE', #6898, .T. ) ;
#11696=CIRCLE ( 'NONE', #10304, 7.500000000000007105 ) ;
#11722=DIRECTION ( 'NONE',  ( -3.061276722312011504E-17, 1.000000000000000000, 0.000000000000000000 ) ) ;
#11743=ORIENTED_EDGE ( 'NONE', *, *, #5405, .F. ) ;
#11825=ADVANCED_FACE ( 'NONE', ( #7608 ), #11373, .T. ) ;
#11879=EDGE_CURVE ( 'NONE', #2829, #6938, #11562, .T. ) ;
#11893=DIRECTION ( 'NONE',  ( 0.000000000000000000, 0.000000000000000000, 1.000000000000000000 ) ) ;
#11940=ORIENTED_EDGE ( 'NONE', *, *, #5993, .F. ) ;
#11957=AXIS2_PLACEMENT_3D ( 'NONE', #9048, #10904, #7955 ) ;
#11966=FACE_BOUND ( 'NONE', #7006, .T. ) ;
#12011=EDGE_LOOP ( 'NONE', ( #1438, #11940, #6503, #11097, #1045 ) ) ;
#12063=ADVANCED_FACE ( 'NONE', ( #10171 ), #4062, .T. ) ;
#12070=EDGE_CURVE ( 'NONE', #867, #481, #7638, .T. ) ;
#12086=CARTESIAN_POINT ( 'NONE',  ( 4.255174644013695128E-15, 25.00000000000002132, -126.4213562373094959 ) ) ;
#12091=VECTOR ( 'NONE', #7859, 1000.000000000000000 ) ;
#12164=DIRECTION ( 'NONE',  ( 0.000000000000000000, 0.000000000000000000, 1.000000000000000000 ) ) ;
#12238=ADVANCED_FACE ( 'NONE', ( #8817 ), #5212, .T. ) ;
ENDSEC;
END-ISO-10303-21;
